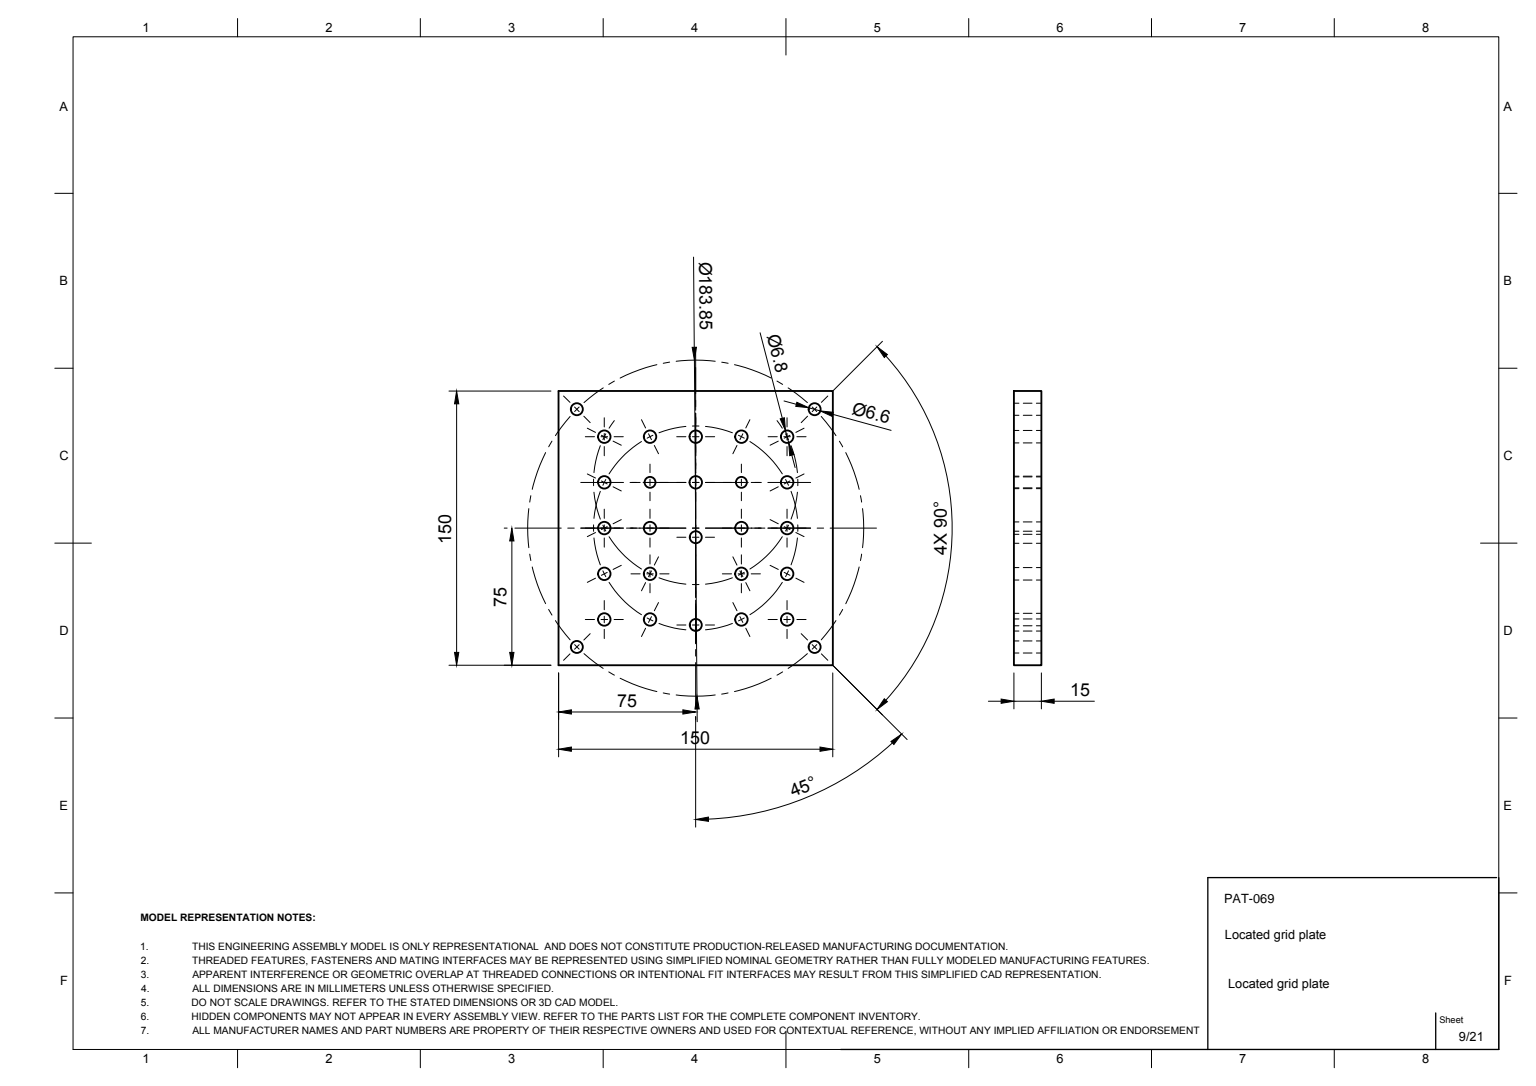
ISO-10303-21;
HEADER;
/* Generated by software containing ST-Developer
 * from STEP Tools, Inc. (www.steptools.com) 
 */

FILE_DESCRIPTION(
/* description */ ('Located fixture plate with toggle clamp'),
/* implementation_level */ '2;1');

FILE_NAME(
/* name */ 'Located grid plate.step',
/* time_stamp */ '2026-10-27T21:36:12-07:00',
/* author */ (''),
/* organization */ (''),
/* preprocessor_version */ 'ST-DEVELOPER v20.2',
/* originating_system */ 'Autodesk Translation Framework v15.17.0.0',
/* authorisation */ '');

FILE_SCHEMA (('AUTOMOTIVE_DESIGN { 1 0 10303 214 3 1 1 }'));
ENDSEC;

DATA;
#10=MECHANICAL_DESIGN_GEOMETRIC_PRESENTATION_REPRESENTATION('',(#325),#9285);
#277=SHAPE_REPRESENTATION_RELATIONSHIP('SRR','None',#9400,#301);
#301=ADVANCED_BREP_SHAPE_REPRESENTATION('',(#348),#9262);
#325=STYLED_ITEM('',(#9598),#348);
#348=MANIFOLD_SOLID_BREP('Body1',#5174);
#388=FACE_BOUND('',#1098,.T.);
#389=FACE_BOUND('',#1099,.T.);
#390=FACE_BOUND('',#1100,.T.);
#391=FACE_BOUND('',#1101,.T.);
#392=FACE_BOUND('',#1102,.T.);
#393=FACE_BOUND('',#1103,.T.);
#394=FACE_BOUND('',#1104,.T.);
#395=FACE_BOUND('',#1105,.T.);
#396=FACE_BOUND('',#1106,.T.);
#397=FACE_BOUND('',#1107,.T.);
#398=FACE_BOUND('',#1108,.T.);
#399=FACE_BOUND('',#1109,.T.);
#400=FACE_BOUND('',#1110,.T.);
#401=FACE_BOUND('',#1111,.T.);
#402=FACE_BOUND('',#1112,.T.);
#403=FACE_BOUND('',#1113,.T.);
#404=FACE_BOUND('',#1114,.T.);
#405=FACE_BOUND('',#1115,.T.);
#406=FACE_BOUND('',#1116,.T.);
#407=FACE_BOUND('',#1117,.T.);
#408=FACE_BOUND('',#1118,.T.);
#409=FACE_BOUND('',#1119,.T.);
#410=FACE_BOUND('',#1120,.T.);
#411=FACE_BOUND('',#1121,.T.);
#412=FACE_BOUND('',#1122,.T.);
#413=FACE_BOUND('',#1123,.T.);
#414=FACE_BOUND('',#1124,.T.);
#415=FACE_BOUND('',#1125,.T.);
#416=FACE_BOUND('',#1128,.T.);
#417=FACE_BOUND('',#1129,.T.);
#418=FACE_BOUND('',#1130,.T.);
#419=FACE_BOUND('',#1131,.T.);
#420=FACE_BOUND('',#1132,.T.);
#421=FACE_BOUND('',#1133,.T.);
#422=FACE_BOUND('',#1134,.T.);
#423=FACE_BOUND('',#1135,.T.);
#424=FACE_BOUND('',#1136,.T.);
#425=FACE_BOUND('',#1137,.T.);
#426=FACE_BOUND('',#1138,.T.);
#427=FACE_BOUND('',#1139,.T.);
#428=FACE_BOUND('',#1140,.T.);
#429=FACE_BOUND('',#1141,.T.);
#430=FACE_BOUND('',#1142,.T.);
#431=FACE_BOUND('',#1143,.T.);
#432=FACE_BOUND('',#1144,.T.);
#433=FACE_BOUND('',#1145,.T.);
#434=FACE_BOUND('',#1146,.T.);
#435=FACE_BOUND('',#1147,.T.);
#436=FACE_BOUND('',#1148,.T.);
#437=FACE_BOUND('',#1149,.T.);
#438=FACE_BOUND('',#1150,.T.);
#439=FACE_BOUND('',#1151,.T.);
#440=FACE_BOUND('',#1152,.T.);
#441=FACE_BOUND('',#1153,.T.);
#442=FACE_BOUND('',#1154,.T.);
#443=FACE_BOUND('',#1155,.T.);
#545=PLANE('',#5666);
#546=PLANE('',#5667);
#547=PLANE('',#5668);
#548=PLANE('',#5669);
#549=PLANE('',#5670);
#550=PLANE('',#5671);
#751=FACE_OUTER_BOUND('',#1068,.T.);
#752=FACE_OUTER_BOUND('',#1069,.T.);
#753=FACE_OUTER_BOUND('',#1070,.T.);
#754=FACE_OUTER_BOUND('',#1071,.T.);
#755=FACE_OUTER_BOUND('',#1072,.T.);
#756=FACE_OUTER_BOUND('',#1073,.T.);
#757=FACE_OUTER_BOUND('',#1074,.T.);
#758=FACE_OUTER_BOUND('',#1075,.T.);
#759=FACE_OUTER_BOUND('',#1076,.T.);
#760=FACE_OUTER_BOUND('',#1077,.T.);
#761=FACE_OUTER_BOUND('',#1078,.T.);
#762=FACE_OUTER_BOUND('',#1079,.T.);
#763=FACE_OUTER_BOUND('',#1080,.T.);
#764=FACE_OUTER_BOUND('',#1081,.T.);
#765=FACE_OUTER_BOUND('',#1082,.T.);
#766=FACE_OUTER_BOUND('',#1083,.T.);
#767=FACE_OUTER_BOUND('',#1084,.T.);
#768=FACE_OUTER_BOUND('',#1085,.T.);
#769=FACE_OUTER_BOUND('',#1086,.T.);
#770=FACE_OUTER_BOUND('',#1087,.T.);
#771=FACE_OUTER_BOUND('',#1088,.T.);
#772=FACE_OUTER_BOUND('',#1089,.T.);
#773=FACE_OUTER_BOUND('',#1090,.T.);
#774=FACE_OUTER_BOUND('',#1091,.T.);
#775=FACE_OUTER_BOUND('',#1092,.T.);
#776=FACE_OUTER_BOUND('',#1093,.T.);
#777=FACE_OUTER_BOUND('',#1094,.T.);
#778=FACE_OUTER_BOUND('',#1095,.T.);
#779=FACE_OUTER_BOUND('',#1096,.T.);
#780=FACE_OUTER_BOUND('',#1097,.T.);
#781=FACE_OUTER_BOUND('',#1126,.T.);
#782=FACE_OUTER_BOUND('',#1127,.T.);
#783=FACE_OUTER_BOUND('',#1156,.T.);
#784=FACE_OUTER_BOUND('',#1157,.T.);
#1068=EDGE_LOOP('',(#3848,#3849,#3850,#3851));
#1069=EDGE_LOOP('',(#3852,#3853,#3854,#3855));
#1070=EDGE_LOOP('',(#3856,#3857,#3858,#3859));
#1071=EDGE_LOOP('',(#3860,#3861,#3862,#3863));
#1072=EDGE_LOOP('',(#3864,#3865,#3866,#3867));
#1073=EDGE_LOOP('',(#3868,#3869,#3870,#3871));
#1074=EDGE_LOOP('',(#3872,#3873,#3874,#3875));
#1075=EDGE_LOOP('',(#3876,#3877,#3878,#3879));
#1076=EDGE_LOOP('',(#3880,#3881,#3882,#3883));
#1077=EDGE_LOOP('',(#3884,#3885,#3886,#3887));
#1078=EDGE_LOOP('',(#3888,#3889,#3890,#3891));
#1079=EDGE_LOOP('',(#3892,#3893,#3894,#3895));
#1080=EDGE_LOOP('',(#3896,#3897,#3898,#3899));
#1081=EDGE_LOOP('',(#3900,#3901,#3902,#3903));
#1082=EDGE_LOOP('',(#3904,#3905,#3906,#3907));
#1083=EDGE_LOOP('',(#3908,#3909,#3910,#3911));
#1084=EDGE_LOOP('',(#3912,#3913,#3914,#3915));
#1085=EDGE_LOOP('',(#3916,#3917,#3918,#3919));
#1086=EDGE_LOOP('',(#3920,#3921,#3922,#3923));
#1087=EDGE_LOOP('',(#3924,#3925,#3926,#3927));
#1088=EDGE_LOOP('',(#3928,#3929,#3930,#3931));
#1089=EDGE_LOOP('',(#3932,#3933,#3934,#3935));
#1090=EDGE_LOOP('',(#3936,#3937,#3938,#3939));
#1091=EDGE_LOOP('',(#3940,#3941,#3942,#3943));
#1092=EDGE_LOOP('',(#3944,#3945,#3946,#3947));
#1093=EDGE_LOOP('',(#3948,#3949,#3950,#3951));
#1094=EDGE_LOOP('',(#3952,#3953,#3954,#3955));
#1095=EDGE_LOOP('',(#3956,#3957,#3958,#3959));
#1096=EDGE_LOOP('',(#3960,#3961,#3962,#3963));
#1097=EDGE_LOOP('',(#3964,#3965,#3966,#3967));
#1098=EDGE_LOOP('',(#3968));
#1099=EDGE_LOOP('',(#3969));
#1100=EDGE_LOOP('',(#3970));
#1101=EDGE_LOOP('',(#3971));
#1102=EDGE_LOOP('',(#3972));
#1103=EDGE_LOOP('',(#3973));
#1104=EDGE_LOOP('',(#3974));
#1105=EDGE_LOOP('',(#3975));
#1106=EDGE_LOOP('',(#3976));
#1107=EDGE_LOOP('',(#3977));
#1108=EDGE_LOOP('',(#3978));
#1109=EDGE_LOOP('',(#3979));
#1110=EDGE_LOOP('',(#3980));
#1111=EDGE_LOOP('',(#3981));
#1112=EDGE_LOOP('',(#3982));
#1113=EDGE_LOOP('',(#3983));
#1114=EDGE_LOOP('',(#3984));
#1115=EDGE_LOOP('',(#3985));
#1116=EDGE_LOOP('',(#3986));
#1117=EDGE_LOOP('',(#3987));
#1118=EDGE_LOOP('',(#3988));
#1119=EDGE_LOOP('',(#3989));
#1120=EDGE_LOOP('',(#3990));
#1121=EDGE_LOOP('',(#3991));
#1122=EDGE_LOOP('',(#3992));
#1123=EDGE_LOOP('',(#3993));
#1124=EDGE_LOOP('',(#3994));
#1125=EDGE_LOOP('',(#3995));
#1126=EDGE_LOOP('',(#3996,#3997,#3998,#3999));
#1127=EDGE_LOOP('',(#4000,#4001,#4002,#4003));
#1128=EDGE_LOOP('',(#4004));
#1129=EDGE_LOOP('',(#4005));
#1130=EDGE_LOOP('',(#4006));
#1131=EDGE_LOOP('',(#4007));
#1132=EDGE_LOOP('',(#4008));
#1133=EDGE_LOOP('',(#4009));
#1134=EDGE_LOOP('',(#4010));
#1135=EDGE_LOOP('',(#4011));
#1136=EDGE_LOOP('',(#4012));
#1137=EDGE_LOOP('',(#4013));
#1138=EDGE_LOOP('',(#4014));
#1139=EDGE_LOOP('',(#4015));
#1140=EDGE_LOOP('',(#4016));
#1141=EDGE_LOOP('',(#4017));
#1142=EDGE_LOOP('',(#4018));
#1143=EDGE_LOOP('',(#4019));
#1144=EDGE_LOOP('',(#4020));
#1145=EDGE_LOOP('',(#4021));
#1146=EDGE_LOOP('',(#4022));
#1147=EDGE_LOOP('',(#4023));
#1148=EDGE_LOOP('',(#4024));
#1149=EDGE_LOOP('',(#4025));
#1150=EDGE_LOOP('',(#4026));
#1151=EDGE_LOOP('',(#4027));
#1152=EDGE_LOOP('',(#4028));
#1153=EDGE_LOOP('',(#4029));
#1154=EDGE_LOOP('',(#4030));
#1155=EDGE_LOOP('',(#4031));
#1156=EDGE_LOOP('',(#4032,#4033,#4034,#4035));
#1157=EDGE_LOOP('',(#4036,#4037,#4038,#4039));
#1419=CIRCLE('',#5583,0.3);
#1420=CIRCLE('',#5584,0.3);
#1421=CIRCLE('',#5586,0.3);
#1422=CIRCLE('',#5587,0.3);
#1423=CIRCLE('',#5589,0.33);
#1424=CIRCLE('',#5590,0.33);
#1425=CIRCLE('',#5592,0.33);
#1426=CIRCLE('',#5593,0.33);
#1427=CIRCLE('',#5595,0.33);
#1428=CIRCLE('',#5596,0.33);
#1429=CIRCLE('',#5598,0.33);
#1430=CIRCLE('',#5599,0.33);
#1431=CIRCLE('',#5601,0.33);
#1432=CIRCLE('',#5602,0.33);
#1433=CIRCLE('',#5604,0.33);
#1434=CIRCLE('',#5605,0.33);
#1435=CIRCLE('',#5607,0.34);
#1436=CIRCLE('',#5608,0.34);
#1437=CIRCLE('',#5610,0.34);
#1438=CIRCLE('',#5611,0.34);
#1439=CIRCLE('',#5613,0.34);
#1440=CIRCLE('',#5614,0.34);
#1441=CIRCLE('',#5616,0.34);
#1442=CIRCLE('',#5617,0.34);
#1443=CIRCLE('',#5619,0.34);
#1444=CIRCLE('',#5620,0.34);
#1445=CIRCLE('',#5622,0.34);
#1446=CIRCLE('',#5623,0.34);
#1447=CIRCLE('',#5625,0.34);
#1448=CIRCLE('',#5626,0.34);
#1449=CIRCLE('',#5628,0.34);
#1450=CIRCLE('',#5629,0.34);
#1451=CIRCLE('',#5631,0.34);
#1452=CIRCLE('',#5632,0.34);
#1453=CIRCLE('',#5634,0.34);
#1454=CIRCLE('',#5635,0.34);
#1455=CIRCLE('',#5637,0.34);
#1456=CIRCLE('',#5638,0.34);
#1457=CIRCLE('',#5640,0.34);
#1458=CIRCLE('',#5641,0.34);
#1459=CIRCLE('',#5643,0.34);
#1460=CIRCLE('',#5644,0.34);
#1461=CIRCLE('',#5646,0.34);
#1462=CIRCLE('',#5647,0.34);
#1463=CIRCLE('',#5649,0.34);
#1464=CIRCLE('',#5650,0.34);
#1465=CIRCLE('',#5652,0.34);
#1466=CIRCLE('',#5653,0.34);
#1467=CIRCLE('',#5655,0.34);
#1468=CIRCLE('',#5656,0.34);
#1469=CIRCLE('',#5658,0.34);
#1470=CIRCLE('',#5659,0.34);
#1471=CIRCLE('',#5661,0.34);
#1472=CIRCLE('',#5662,0.34);
#1473=CIRCLE('',#5664,0.34);
#1474=CIRCLE('',#5665,0.34);
#1727=LINE('',#7966,#2137);
#1728=LINE('',#7972,#2138);
#1729=LINE('',#7978,#2139);
#1730=LINE('',#7984,#2140);
#1731=LINE('',#7990,#2141);
#1732=LINE('',#7996,#2142);
#1733=LINE('',#8002,#2143);
#1734=LINE('',#8008,#2144);
#1735=LINE('',#8014,#2145);
#1736=LINE('',#8020,#2146);
#1737=LINE('',#8026,#2147);
#1738=LINE('',#8032,#2148);
#1739=LINE('',#8038,#2149);
#1740=LINE('',#8044,#2150);
#1741=LINE('',#8050,#2151);
#1742=LINE('',#8056,#2152);
#1743=LINE('',#8062,#2153);
#1744=LINE('',#8068,#2154);
#1745=LINE('',#8074,#2155);
#1746=LINE('',#8080,#2156);
#1747=LINE('',#8086,#2157);
#1748=LINE('',#8092,#2158);
#1749=LINE('',#8098,#2159);
#1750=LINE('',#8104,#2160);
#1751=LINE('',#8110,#2161);
#1752=LINE('',#8116,#2162);
#1753=LINE('',#8122,#2163);
#1754=LINE('',#8128,#2164);
#1755=LINE('',#8133,#2165);
#1756=LINE('',#8135,#2166);
#1757=LINE('',#8137,#2167);
#1758=LINE('',#8138,#2168);
#1759=LINE('',#8141,#2169);
#1760=LINE('',#8143,#2170);
#1761=LINE('',#8144,#2171);
#1762=LINE('',#8147,#2172);
#1763=LINE('',#8149,#2173);
#1764=LINE('',#8150,#2174);
#1765=LINE('',#8152,#2175);
#1766=LINE('',#8153,#2176);
#2137=VECTOR('',#6421,0.3);
#2138=VECTOR('',#6428,0.3);
#2139=VECTOR('',#6435,0.33);
#2140=VECTOR('',#6442,0.33);
#2141=VECTOR('',#6449,0.33);
#2142=VECTOR('',#6456,0.33);
#2143=VECTOR('',#6463,0.33);
#2144=VECTOR('',#6470,0.33);
#2145=VECTOR('',#6477,0.34);
#2146=VECTOR('',#6484,0.34);
#2147=VECTOR('',#6491,0.34);
#2148=VECTOR('',#6498,0.34);
#2149=VECTOR('',#6505,0.34);
#2150=VECTOR('',#6512,0.34);
#2151=VECTOR('',#6519,0.34);
#2152=VECTOR('',#6526,0.34);
#2153=VECTOR('',#6533,0.34);
#2154=VECTOR('',#6540,0.34);
#2155=VECTOR('',#6547,0.34);
#2156=VECTOR('',#6554,0.34);
#2157=VECTOR('',#6561,0.34);
#2158=VECTOR('',#6568,0.34);
#2159=VECTOR('',#6575,0.34);
#2160=VECTOR('',#6582,0.34);
#2161=VECTOR('',#6589,0.34);
#2162=VECTOR('',#6596,0.34);
#2163=VECTOR('',#6603,0.34);
#2164=VECTOR('',#6610,0.34);
#2165=VECTOR('',#6615,1.);
#2166=VECTOR('',#6616,1.);
#2167=VECTOR('',#6617,1.);
#2168=VECTOR('',#6618,1.);
#2169=VECTOR('',#6621,1.);
#2170=VECTOR('',#6622,1.);
#2171=VECTOR('',#6623,1.);
#2172=VECTOR('',#6626,1.);
#2173=VECTOR('',#6627,1.);
#2174=VECTOR('',#6628,1.);
#2175=VECTOR('',#6631,1.);
#2176=VECTOR('',#6632,1.);
#2521=VERTEX_POINT('',#7963);
#2522=VERTEX_POINT('',#7965);
#2523=VERTEX_POINT('',#7969);
#2524=VERTEX_POINT('',#7971);
#2525=VERTEX_POINT('',#7975);
#2526=VERTEX_POINT('',#7977);
#2527=VERTEX_POINT('',#7981);
#2528=VERTEX_POINT('',#7983);
#2529=VERTEX_POINT('',#7987);
#2530=VERTEX_POINT('',#7989);
#2531=VERTEX_POINT('',#7993);
#2532=VERTEX_POINT('',#7995);
#2533=VERTEX_POINT('',#7999);
#2534=VERTEX_POINT('',#8001);
#2535=VERTEX_POINT('',#8005);
#2536=VERTEX_POINT('',#8007);
#2537=VERTEX_POINT('',#8011);
#2538=VERTEX_POINT('',#8013);
#2539=VERTEX_POINT('',#8017);
#2540=VERTEX_POINT('',#8019);
#2541=VERTEX_POINT('',#8023);
#2542=VERTEX_POINT('',#8025);
#2543=VERTEX_POINT('',#8029);
#2544=VERTEX_POINT('',#8031);
#2545=VERTEX_POINT('',#8035);
#2546=VERTEX_POINT('',#8037);
#2547=VERTEX_POINT('',#8041);
#2548=VERTEX_POINT('',#8043);
#2549=VERTEX_POINT('',#8047);
#2550=VERTEX_POINT('',#8049);
#2551=VERTEX_POINT('',#8053);
#2552=VERTEX_POINT('',#8055);
#2553=VERTEX_POINT('',#8059);
#2554=VERTEX_POINT('',#8061);
#2555=VERTEX_POINT('',#8065);
#2556=VERTEX_POINT('',#8067);
#2557=VERTEX_POINT('',#8071);
#2558=VERTEX_POINT('',#8073);
#2559=VERTEX_POINT('',#8077);
#2560=VERTEX_POINT('',#8079);
#2561=VERTEX_POINT('',#8083);
#2562=VERTEX_POINT('',#8085);
#2563=VERTEX_POINT('',#8089);
#2564=VERTEX_POINT('',#8091);
#2565=VERTEX_POINT('',#8095);
#2566=VERTEX_POINT('',#8097);
#2567=VERTEX_POINT('',#8101);
#2568=VERTEX_POINT('',#8103);
#2569=VERTEX_POINT('',#8107);
#2570=VERTEX_POINT('',#8109);
#2571=VERTEX_POINT('',#8113);
#2572=VERTEX_POINT('',#8115);
#2573=VERTEX_POINT('',#8119);
#2574=VERTEX_POINT('',#8121);
#2575=VERTEX_POINT('',#8125);
#2576=VERTEX_POINT('',#8127);
#2577=VERTEX_POINT('',#8131);
#2578=VERTEX_POINT('',#8132);
#2579=VERTEX_POINT('',#8134);
#2580=VERTEX_POINT('',#8136);
#2581=VERTEX_POINT('',#8140);
#2582=VERTEX_POINT('',#8142);
#2583=VERTEX_POINT('',#8146);
#2584=VERTEX_POINT('',#8148);
#3012=EDGE_CURVE('',#2521,#2521,#1419,.T.);
#3013=EDGE_CURVE('',#2521,#2522,#1727,.T.);
#3014=EDGE_CURVE('',#2522,#2522,#1420,.T.);
#3015=EDGE_CURVE('',#2523,#2523,#1421,.T.);
#3016=EDGE_CURVE('',#2523,#2524,#1728,.T.);
#3017=EDGE_CURVE('',#2524,#2524,#1422,.T.);
#3018=EDGE_CURVE('',#2525,#2525,#1423,.T.);
#3019=EDGE_CURVE('',#2525,#2526,#1729,.T.);
#3020=EDGE_CURVE('',#2526,#2526,#1424,.T.);
#3021=EDGE_CURVE('',#2527,#2527,#1425,.T.);
#3022=EDGE_CURVE('',#2527,#2528,#1730,.T.);
#3023=EDGE_CURVE('',#2528,#2528,#1426,.T.);
#3024=EDGE_CURVE('',#2529,#2529,#1427,.T.);
#3025=EDGE_CURVE('',#2529,#2530,#1731,.T.);
#3026=EDGE_CURVE('',#2530,#2530,#1428,.T.);
#3027=EDGE_CURVE('',#2531,#2531,#1429,.T.);
#3028=EDGE_CURVE('',#2531,#2532,#1732,.T.);
#3029=EDGE_CURVE('',#2532,#2532,#1430,.T.);
#3030=EDGE_CURVE('',#2533,#2533,#1431,.T.);
#3031=EDGE_CURVE('',#2533,#2534,#1733,.T.);
#3032=EDGE_CURVE('',#2534,#2534,#1432,.T.);
#3033=EDGE_CURVE('',#2535,#2535,#1433,.T.);
#3034=EDGE_CURVE('',#2535,#2536,#1734,.T.);
#3035=EDGE_CURVE('',#2536,#2536,#1434,.T.);
#3036=EDGE_CURVE('',#2537,#2537,#1435,.T.);
#3037=EDGE_CURVE('',#2537,#2538,#1735,.T.);
#3038=EDGE_CURVE('',#2538,#2538,#1436,.T.);
#3039=EDGE_CURVE('',#2539,#2539,#1437,.T.);
#3040=EDGE_CURVE('',#2539,#2540,#1736,.T.);
#3041=EDGE_CURVE('',#2540,#2540,#1438,.T.);
#3042=EDGE_CURVE('',#2541,#2541,#1439,.T.);
#3043=EDGE_CURVE('',#2541,#2542,#1737,.T.);
#3044=EDGE_CURVE('',#2542,#2542,#1440,.T.);
#3045=EDGE_CURVE('',#2543,#2543,#1441,.T.);
#3046=EDGE_CURVE('',#2543,#2544,#1738,.T.);
#3047=EDGE_CURVE('',#2544,#2544,#1442,.T.);
#3048=EDGE_CURVE('',#2545,#2545,#1443,.T.);
#3049=EDGE_CURVE('',#2545,#2546,#1739,.T.);
#3050=EDGE_CURVE('',#2546,#2546,#1444,.T.);
#3051=EDGE_CURVE('',#2547,#2547,#1445,.T.);
#3052=EDGE_CURVE('',#2547,#2548,#1740,.T.);
#3053=EDGE_CURVE('',#2548,#2548,#1446,.T.);
#3054=EDGE_CURVE('',#2549,#2549,#1447,.T.);
#3055=EDGE_CURVE('',#2549,#2550,#1741,.T.);
#3056=EDGE_CURVE('',#2550,#2550,#1448,.T.);
#3057=EDGE_CURVE('',#2551,#2551,#1449,.T.);
#3058=EDGE_CURVE('',#2551,#2552,#1742,.T.);
#3059=EDGE_CURVE('',#2552,#2552,#1450,.T.);
#3060=EDGE_CURVE('',#2553,#2553,#1451,.T.);
#3061=EDGE_CURVE('',#2553,#2554,#1743,.T.);
#3062=EDGE_CURVE('',#2554,#2554,#1452,.T.);
#3063=EDGE_CURVE('',#2555,#2555,#1453,.T.);
#3064=EDGE_CURVE('',#2555,#2556,#1744,.T.);
#3065=EDGE_CURVE('',#2556,#2556,#1454,.T.);
#3066=EDGE_CURVE('',#2557,#2557,#1455,.T.);
#3067=EDGE_CURVE('',#2557,#2558,#1745,.T.);
#3068=EDGE_CURVE('',#2558,#2558,#1456,.T.);
#3069=EDGE_CURVE('',#2559,#2559,#1457,.T.);
#3070=EDGE_CURVE('',#2559,#2560,#1746,.T.);
#3071=EDGE_CURVE('',#2560,#2560,#1458,.T.);
#3072=EDGE_CURVE('',#2561,#2561,#1459,.T.);
#3073=EDGE_CURVE('',#2561,#2562,#1747,.T.);
#3074=EDGE_CURVE('',#2562,#2562,#1460,.T.);
#3075=EDGE_CURVE('',#2563,#2563,#1461,.T.);
#3076=EDGE_CURVE('',#2563,#2564,#1748,.T.);
#3077=EDGE_CURVE('',#2564,#2564,#1462,.T.);
#3078=EDGE_CURVE('',#2565,#2565,#1463,.T.);
#3079=EDGE_CURVE('',#2565,#2566,#1749,.T.);
#3080=EDGE_CURVE('',#2566,#2566,#1464,.T.);
#3081=EDGE_CURVE('',#2567,#2567,#1465,.T.);
#3082=EDGE_CURVE('',#2567,#2568,#1750,.T.);
#3083=EDGE_CURVE('',#2568,#2568,#1466,.T.);
#3084=EDGE_CURVE('',#2569,#2569,#1467,.T.);
#3085=EDGE_CURVE('',#2569,#2570,#1751,.T.);
#3086=EDGE_CURVE('',#2570,#2570,#1468,.T.);
#3087=EDGE_CURVE('',#2571,#2571,#1469,.T.);
#3088=EDGE_CURVE('',#2571,#2572,#1752,.T.);
#3089=EDGE_CURVE('',#2572,#2572,#1470,.T.);
#3090=EDGE_CURVE('',#2573,#2573,#1471,.T.);
#3091=EDGE_CURVE('',#2573,#2574,#1753,.T.);
#3092=EDGE_CURVE('',#2574,#2574,#1472,.T.);
#3093=EDGE_CURVE('',#2575,#2575,#1473,.T.);
#3094=EDGE_CURVE('',#2575,#2576,#1754,.T.);
#3095=EDGE_CURVE('',#2576,#2576,#1474,.T.);
#3096=EDGE_CURVE('',#2577,#2578,#1755,.T.);
#3097=EDGE_CURVE('',#2578,#2579,#1756,.T.);
#3098=EDGE_CURVE('',#2580,#2579,#1757,.T.);
#3099=EDGE_CURVE('',#2577,#2580,#1758,.T.);
#3100=EDGE_CURVE('',#2581,#2577,#1759,.T.);
#3101=EDGE_CURVE('',#2582,#2580,#1760,.T.);
#3102=EDGE_CURVE('',#2581,#2582,#1761,.T.);
#3103=EDGE_CURVE('',#2583,#2581,#1762,.T.);
#3104=EDGE_CURVE('',#2584,#2582,#1763,.T.);
#3105=EDGE_CURVE('',#2583,#2584,#1764,.T.);
#3106=EDGE_CURVE('',#2578,#2583,#1765,.T.);
#3107=EDGE_CURVE('',#2579,#2584,#1766,.T.);
#3848=ORIENTED_EDGE('',*,*,#3012,.F.);
#3849=ORIENTED_EDGE('',*,*,#3013,.T.);
#3850=ORIENTED_EDGE('',*,*,#3014,.F.);
#3851=ORIENTED_EDGE('',*,*,#3013,.F.);
#3852=ORIENTED_EDGE('',*,*,#3015,.F.);
#3853=ORIENTED_EDGE('',*,*,#3016,.T.);
#3854=ORIENTED_EDGE('',*,*,#3017,.F.);
#3855=ORIENTED_EDGE('',*,*,#3016,.F.);
#3856=ORIENTED_EDGE('',*,*,#3018,.F.);
#3857=ORIENTED_EDGE('',*,*,#3019,.T.);
#3858=ORIENTED_EDGE('',*,*,#3020,.F.);
#3859=ORIENTED_EDGE('',*,*,#3019,.F.);
#3860=ORIENTED_EDGE('',*,*,#3021,.F.);
#3861=ORIENTED_EDGE('',*,*,#3022,.T.);
#3862=ORIENTED_EDGE('',*,*,#3023,.F.);
#3863=ORIENTED_EDGE('',*,*,#3022,.F.);
#3864=ORIENTED_EDGE('',*,*,#3024,.F.);
#3865=ORIENTED_EDGE('',*,*,#3025,.T.);
#3866=ORIENTED_EDGE('',*,*,#3026,.F.);
#3867=ORIENTED_EDGE('',*,*,#3025,.F.);
#3868=ORIENTED_EDGE('',*,*,#3027,.F.);
#3869=ORIENTED_EDGE('',*,*,#3028,.T.);
#3870=ORIENTED_EDGE('',*,*,#3029,.F.);
#3871=ORIENTED_EDGE('',*,*,#3028,.F.);
#3872=ORIENTED_EDGE('',*,*,#3030,.F.);
#3873=ORIENTED_EDGE('',*,*,#3031,.T.);
#3874=ORIENTED_EDGE('',*,*,#3032,.F.);
#3875=ORIENTED_EDGE('',*,*,#3031,.F.);
#3876=ORIENTED_EDGE('',*,*,#3033,.F.);
#3877=ORIENTED_EDGE('',*,*,#3034,.T.);
#3878=ORIENTED_EDGE('',*,*,#3035,.F.);
#3879=ORIENTED_EDGE('',*,*,#3034,.F.);
#3880=ORIENTED_EDGE('',*,*,#3036,.F.);
#3881=ORIENTED_EDGE('',*,*,#3037,.T.);
#3882=ORIENTED_EDGE('',*,*,#3038,.F.);
#3883=ORIENTED_EDGE('',*,*,#3037,.F.);
#3884=ORIENTED_EDGE('',*,*,#3039,.F.);
#3885=ORIENTED_EDGE('',*,*,#3040,.T.);
#3886=ORIENTED_EDGE('',*,*,#3041,.F.);
#3887=ORIENTED_EDGE('',*,*,#3040,.F.);
#3888=ORIENTED_EDGE('',*,*,#3042,.F.);
#3889=ORIENTED_EDGE('',*,*,#3043,.T.);
#3890=ORIENTED_EDGE('',*,*,#3044,.F.);
#3891=ORIENTED_EDGE('',*,*,#3043,.F.);
#3892=ORIENTED_EDGE('',*,*,#3045,.F.);
#3893=ORIENTED_EDGE('',*,*,#3046,.T.);
#3894=ORIENTED_EDGE('',*,*,#3047,.F.);
#3895=ORIENTED_EDGE('',*,*,#3046,.F.);
#3896=ORIENTED_EDGE('',*,*,#3048,.F.);
#3897=ORIENTED_EDGE('',*,*,#3049,.T.);
#3898=ORIENTED_EDGE('',*,*,#3050,.F.);
#3899=ORIENTED_EDGE('',*,*,#3049,.F.);
#3900=ORIENTED_EDGE('',*,*,#3051,.F.);
#3901=ORIENTED_EDGE('',*,*,#3052,.T.);
#3902=ORIENTED_EDGE('',*,*,#3053,.F.);
#3903=ORIENTED_EDGE('',*,*,#3052,.F.);
#3904=ORIENTED_EDGE('',*,*,#3054,.F.);
#3905=ORIENTED_EDGE('',*,*,#3055,.T.);
#3906=ORIENTED_EDGE('',*,*,#3056,.F.);
#3907=ORIENTED_EDGE('',*,*,#3055,.F.);
#3908=ORIENTED_EDGE('',*,*,#3057,.F.);
#3909=ORIENTED_EDGE('',*,*,#3058,.T.);
#3910=ORIENTED_EDGE('',*,*,#3059,.F.);
#3911=ORIENTED_EDGE('',*,*,#3058,.F.);
#3912=ORIENTED_EDGE('',*,*,#3060,.F.);
#3913=ORIENTED_EDGE('',*,*,#3061,.T.);
#3914=ORIENTED_EDGE('',*,*,#3062,.F.);
#3915=ORIENTED_EDGE('',*,*,#3061,.F.);
#3916=ORIENTED_EDGE('',*,*,#3063,.F.);
#3917=ORIENTED_EDGE('',*,*,#3064,.T.);
#3918=ORIENTED_EDGE('',*,*,#3065,.F.);
#3919=ORIENTED_EDGE('',*,*,#3064,.F.);
#3920=ORIENTED_EDGE('',*,*,#3066,.F.);
#3921=ORIENTED_EDGE('',*,*,#3067,.T.);
#3922=ORIENTED_EDGE('',*,*,#3068,.F.);
#3923=ORIENTED_EDGE('',*,*,#3067,.F.);
#3924=ORIENTED_EDGE('',*,*,#3069,.F.);
#3925=ORIENTED_EDGE('',*,*,#3070,.T.);
#3926=ORIENTED_EDGE('',*,*,#3071,.F.);
#3927=ORIENTED_EDGE('',*,*,#3070,.F.);
#3928=ORIENTED_EDGE('',*,*,#3072,.F.);
#3929=ORIENTED_EDGE('',*,*,#3073,.T.);
#3930=ORIENTED_EDGE('',*,*,#3074,.F.);
#3931=ORIENTED_EDGE('',*,*,#3073,.F.);
#3932=ORIENTED_EDGE('',*,*,#3075,.F.);
#3933=ORIENTED_EDGE('',*,*,#3076,.T.);
#3934=ORIENTED_EDGE('',*,*,#3077,.F.);
#3935=ORIENTED_EDGE('',*,*,#3076,.F.);
#3936=ORIENTED_EDGE('',*,*,#3078,.F.);
#3937=ORIENTED_EDGE('',*,*,#3079,.T.);
#3938=ORIENTED_EDGE('',*,*,#3080,.F.);
#3939=ORIENTED_EDGE('',*,*,#3079,.F.);
#3940=ORIENTED_EDGE('',*,*,#3081,.F.);
#3941=ORIENTED_EDGE('',*,*,#3082,.T.);
#3942=ORIENTED_EDGE('',*,*,#3083,.F.);
#3943=ORIENTED_EDGE('',*,*,#3082,.F.);
#3944=ORIENTED_EDGE('',*,*,#3084,.F.);
#3945=ORIENTED_EDGE('',*,*,#3085,.T.);
#3946=ORIENTED_EDGE('',*,*,#3086,.F.);
#3947=ORIENTED_EDGE('',*,*,#3085,.F.);
#3948=ORIENTED_EDGE('',*,*,#3087,.F.);
#3949=ORIENTED_EDGE('',*,*,#3088,.T.);
#3950=ORIENTED_EDGE('',*,*,#3089,.F.);
#3951=ORIENTED_EDGE('',*,*,#3088,.F.);
#3952=ORIENTED_EDGE('',*,*,#3090,.F.);
#3953=ORIENTED_EDGE('',*,*,#3091,.T.);
#3954=ORIENTED_EDGE('',*,*,#3092,.F.);
#3955=ORIENTED_EDGE('',*,*,#3091,.F.);
#3956=ORIENTED_EDGE('',*,*,#3093,.F.);
#3957=ORIENTED_EDGE('',*,*,#3094,.T.);
#3958=ORIENTED_EDGE('',*,*,#3095,.F.);
#3959=ORIENTED_EDGE('',*,*,#3094,.F.);
#3960=ORIENTED_EDGE('',*,*,#3096,.T.);
#3961=ORIENTED_EDGE('',*,*,#3097,.T.);
#3962=ORIENTED_EDGE('',*,*,#3098,.F.);
#3963=ORIENTED_EDGE('',*,*,#3099,.F.);
#3964=ORIENTED_EDGE('',*,*,#3100,.T.);
#3965=ORIENTED_EDGE('',*,*,#3099,.T.);
#3966=ORIENTED_EDGE('',*,*,#3101,.F.);
#3967=ORIENTED_EDGE('',*,*,#3102,.F.);
#3968=ORIENTED_EDGE('',*,*,#3020,.T.);
#3969=ORIENTED_EDGE('',*,*,#3023,.T.);
#3970=ORIENTED_EDGE('',*,*,#3026,.T.);
#3971=ORIENTED_EDGE('',*,*,#3029,.T.);
#3972=ORIENTED_EDGE('',*,*,#3038,.T.);
#3973=ORIENTED_EDGE('',*,*,#3041,.T.);
#3974=ORIENTED_EDGE('',*,*,#3044,.T.);
#3975=ORIENTED_EDGE('',*,*,#3047,.T.);
#3976=ORIENTED_EDGE('',*,*,#3050,.T.);
#3977=ORIENTED_EDGE('',*,*,#3053,.T.);
#3978=ORIENTED_EDGE('',*,*,#3056,.T.);
#3979=ORIENTED_EDGE('',*,*,#3059,.T.);
#3980=ORIENTED_EDGE('',*,*,#3062,.T.);
#3981=ORIENTED_EDGE('',*,*,#3065,.T.);
#3982=ORIENTED_EDGE('',*,*,#3068,.T.);
#3983=ORIENTED_EDGE('',*,*,#3071,.T.);
#3984=ORIENTED_EDGE('',*,*,#3074,.T.);
#3985=ORIENTED_EDGE('',*,*,#3077,.T.);
#3986=ORIENTED_EDGE('',*,*,#3080,.T.);
#3987=ORIENTED_EDGE('',*,*,#3083,.T.);
#3988=ORIENTED_EDGE('',*,*,#3086,.T.);
#3989=ORIENTED_EDGE('',*,*,#3089,.T.);
#3990=ORIENTED_EDGE('',*,*,#3092,.T.);
#3991=ORIENTED_EDGE('',*,*,#3095,.T.);
#3992=ORIENTED_EDGE('',*,*,#3035,.T.);
#3993=ORIENTED_EDGE('',*,*,#3032,.T.);
#3994=ORIENTED_EDGE('',*,*,#3017,.T.);
#3995=ORIENTED_EDGE('',*,*,#3014,.T.);
#3996=ORIENTED_EDGE('',*,*,#3103,.T.);
#3997=ORIENTED_EDGE('',*,*,#3102,.T.);
#3998=ORIENTED_EDGE('',*,*,#3104,.F.);
#3999=ORIENTED_EDGE('',*,*,#3105,.F.);
#4000=ORIENTED_EDGE('',*,*,#3106,.T.);
#4001=ORIENTED_EDGE('',*,*,#3105,.T.);
#4002=ORIENTED_EDGE('',*,*,#3107,.F.);
#4003=ORIENTED_EDGE('',*,*,#3097,.F.);
#4004=ORIENTED_EDGE('',*,*,#3018,.T.);
#4005=ORIENTED_EDGE('',*,*,#3021,.T.);
#4006=ORIENTED_EDGE('',*,*,#3024,.T.);
#4007=ORIENTED_EDGE('',*,*,#3027,.T.);
#4008=ORIENTED_EDGE('',*,*,#3036,.T.);
#4009=ORIENTED_EDGE('',*,*,#3039,.T.);
#4010=ORIENTED_EDGE('',*,*,#3042,.T.);
#4011=ORIENTED_EDGE('',*,*,#3045,.T.);
#4012=ORIENTED_EDGE('',*,*,#3048,.T.);
#4013=ORIENTED_EDGE('',*,*,#3051,.T.);
#4014=ORIENTED_EDGE('',*,*,#3054,.T.);
#4015=ORIENTED_EDGE('',*,*,#3057,.T.);
#4016=ORIENTED_EDGE('',*,*,#3060,.T.);
#4017=ORIENTED_EDGE('',*,*,#3063,.T.);
#4018=ORIENTED_EDGE('',*,*,#3066,.T.);
#4019=ORIENTED_EDGE('',*,*,#3069,.T.);
#4020=ORIENTED_EDGE('',*,*,#3072,.T.);
#4021=ORIENTED_EDGE('',*,*,#3075,.T.);
#4022=ORIENTED_EDGE('',*,*,#3078,.T.);
#4023=ORIENTED_EDGE('',*,*,#3081,.T.);
#4024=ORIENTED_EDGE('',*,*,#3084,.T.);
#4025=ORIENTED_EDGE('',*,*,#3087,.T.);
#4026=ORIENTED_EDGE('',*,*,#3090,.T.);
#4027=ORIENTED_EDGE('',*,*,#3093,.T.);
#4028=ORIENTED_EDGE('',*,*,#3033,.T.);
#4029=ORIENTED_EDGE('',*,*,#3030,.T.);
#4030=ORIENTED_EDGE('',*,*,#3015,.T.);
#4031=ORIENTED_EDGE('',*,*,#3012,.T.);
#4032=ORIENTED_EDGE('',*,*,#3107,.T.);
#4033=ORIENTED_EDGE('',*,*,#3104,.T.);
#4034=ORIENTED_EDGE('',*,*,#3101,.T.);
#4035=ORIENTED_EDGE('',*,*,#3098,.T.);
#4036=ORIENTED_EDGE('',*,*,#3106,.F.);
#4037=ORIENTED_EDGE('',*,*,#3096,.F.);
#4038=ORIENTED_EDGE('',*,*,#3100,.F.);
#4039=ORIENTED_EDGE('',*,*,#3103,.F.);
#4807=CYLINDRICAL_SURFACE('',#5582,0.3);
#4808=CYLINDRICAL_SURFACE('',#5585,0.3);
#4809=CYLINDRICAL_SURFACE('',#5588,0.33);
#4810=CYLINDRICAL_SURFACE('',#5591,0.33);
#4811=CYLINDRICAL_SURFACE('',#5594,0.33);
#4812=CYLINDRICAL_SURFACE('',#5597,0.33);
#4813=CYLINDRICAL_SURFACE('',#5600,0.33);
#4814=CYLINDRICAL_SURFACE('',#5603,0.33);
#4815=CYLINDRICAL_SURFACE('',#5606,0.34);
#4816=CYLINDRICAL_SURFACE('',#5609,0.34);
#4817=CYLINDRICAL_SURFACE('',#5612,0.34);
#4818=CYLINDRICAL_SURFACE('',#5615,0.34);
#4819=CYLINDRICAL_SURFACE('',#5618,0.34);
#4820=CYLINDRICAL_SURFACE('',#5621,0.34);
#4821=CYLINDRICAL_SURFACE('',#5624,0.34);
#4822=CYLINDRICAL_SURFACE('',#5627,0.34);
#4823=CYLINDRICAL_SURFACE('',#5630,0.34);
#4824=CYLINDRICAL_SURFACE('',#5633,0.34);
#4825=CYLINDRICAL_SURFACE('',#5636,0.34);
#4826=CYLINDRICAL_SURFACE('',#5639,0.34);
#4827=CYLINDRICAL_SURFACE('',#5642,0.34);
#4828=CYLINDRICAL_SURFACE('',#5645,0.34);
#4829=CYLINDRICAL_SURFACE('',#5648,0.34);
#4830=CYLINDRICAL_SURFACE('',#5651,0.34);
#4831=CYLINDRICAL_SURFACE('',#5654,0.34);
#4832=CYLINDRICAL_SURFACE('',#5657,0.34);
#4833=CYLINDRICAL_SURFACE('',#5660,0.34);
#4834=CYLINDRICAL_SURFACE('',#5663,0.34);
#4952=ADVANCED_FACE('',(#751),#4807,.F.);
#4953=ADVANCED_FACE('',(#752),#4808,.F.);
#4954=ADVANCED_FACE('',(#753),#4809,.F.);
#4955=ADVANCED_FACE('',(#754),#4810,.F.);
#4956=ADVANCED_FACE('',(#755),#4811,.F.);
#4957=ADVANCED_FACE('',(#756),#4812,.F.);
#4958=ADVANCED_FACE('',(#757),#4813,.F.);
#4959=ADVANCED_FACE('',(#758),#4814,.F.);
#4960=ADVANCED_FACE('',(#759),#4815,.F.);
#4961=ADVANCED_FACE('',(#760),#4816,.F.);
#4962=ADVANCED_FACE('',(#761),#4817,.F.);
#4963=ADVANCED_FACE('',(#762),#4818,.F.);
#4964=ADVANCED_FACE('',(#763),#4819,.F.);
#4965=ADVANCED_FACE('',(#764),#4820,.F.);
#4966=ADVANCED_FACE('',(#765),#4821,.F.);
#4967=ADVANCED_FACE('',(#766),#4822,.F.);
#4968=ADVANCED_FACE('',(#767),#4823,.F.);
#4969=ADVANCED_FACE('',(#768),#4824,.F.);
#4970=ADVANCED_FACE('',(#769),#4825,.F.);
#4971=ADVANCED_FACE('',(#770),#4826,.F.);
#4972=ADVANCED_FACE('',(#771),#4827,.F.);
#4973=ADVANCED_FACE('',(#772),#4828,.F.);
#4974=ADVANCED_FACE('',(#773),#4829,.F.);
#4975=ADVANCED_FACE('',(#774),#4830,.F.);
#4976=ADVANCED_FACE('',(#775),#4831,.F.);
#4977=ADVANCED_FACE('',(#776),#4832,.F.);
#4978=ADVANCED_FACE('',(#777),#4833,.F.);
#4979=ADVANCED_FACE('',(#778),#4834,.F.);
#4980=ADVANCED_FACE('',(#779),#545,.T.);
#4981=ADVANCED_FACE('',(#780,#388,#389,#390,#391,#392,#393,#394,#395,#396,
#397,#398,#399,#400,#401,#402,#403,#404,#405,#406,#407,#408,#409,#410,#411,
#412,#413,#414,#415),#546,.T.);
#4982=ADVANCED_FACE('',(#781),#547,.T.);
#4983=ADVANCED_FACE('',(#782,#416,#417,#418,#419,#420,#421,#422,#423,#424,
#425,#426,#427,#428,#429,#430,#431,#432,#433,#434,#435,#436,#437,#438,#439,
#440,#441,#442,#443),#548,.T.);
#4984=ADVANCED_FACE('',(#783),#549,.T.);
#4985=ADVANCED_FACE('',(#784),#550,.F.);
#5174=CLOSED_SHELL('',(#4952,#4953,#4954,#4955,#4956,#4957,#4958,#4959,
#4960,#4961,#4962,#4963,#4964,#4965,#4966,#4967,#4968,#4969,#4970,#4971,
#4972,#4973,#4974,#4975,#4976,#4977,#4978,#4979,#4980,#4981,#4982,#4983,
#4984,#4985));
#5581=AXIS2_PLACEMENT_3D('',#7961,#6415,#6416);
#5582=AXIS2_PLACEMENT_3D('',#7962,#6417,#6418);
#5583=AXIS2_PLACEMENT_3D('',#7964,#6419,#6420);
#5584=AXIS2_PLACEMENT_3D('',#7967,#6422,#6423);
#5585=AXIS2_PLACEMENT_3D('',#7968,#6424,#6425);
#5586=AXIS2_PLACEMENT_3D('',#7970,#6426,#6427);
#5587=AXIS2_PLACEMENT_3D('',#7973,#6429,#6430);
#5588=AXIS2_PLACEMENT_3D('',#7974,#6431,#6432);
#5589=AXIS2_PLACEMENT_3D('',#7976,#6433,#6434);
#5590=AXIS2_PLACEMENT_3D('',#7979,#6436,#6437);
#5591=AXIS2_PLACEMENT_3D('',#7980,#6438,#6439);
#5592=AXIS2_PLACEMENT_3D('',#7982,#6440,#6441);
#5593=AXIS2_PLACEMENT_3D('',#7985,#6443,#6444);
#5594=AXIS2_PLACEMENT_3D('',#7986,#6445,#6446);
#5595=AXIS2_PLACEMENT_3D('',#7988,#6447,#6448);
#5596=AXIS2_PLACEMENT_3D('',#7991,#6450,#6451);
#5597=AXIS2_PLACEMENT_3D('',#7992,#6452,#6453);
#5598=AXIS2_PLACEMENT_3D('',#7994,#6454,#6455);
#5599=AXIS2_PLACEMENT_3D('',#7997,#6457,#6458);
#5600=AXIS2_PLACEMENT_3D('',#7998,#6459,#6460);
#5601=AXIS2_PLACEMENT_3D('',#8000,#6461,#6462);
#5602=AXIS2_PLACEMENT_3D('',#8003,#6464,#6465);
#5603=AXIS2_PLACEMENT_3D('',#8004,#6466,#6467);
#5604=AXIS2_PLACEMENT_3D('',#8006,#6468,#6469);
#5605=AXIS2_PLACEMENT_3D('',#8009,#6471,#6472);
#5606=AXIS2_PLACEMENT_3D('',#8010,#6473,#6474);
#5607=AXIS2_PLACEMENT_3D('',#8012,#6475,#6476);
#5608=AXIS2_PLACEMENT_3D('',#8015,#6478,#6479);
#5609=AXIS2_PLACEMENT_3D('',#8016,#6480,#6481);
#5610=AXIS2_PLACEMENT_3D('',#8018,#6482,#6483);
#5611=AXIS2_PLACEMENT_3D('',#8021,#6485,#6486);
#5612=AXIS2_PLACEMENT_3D('',#8022,#6487,#6488);
#5613=AXIS2_PLACEMENT_3D('',#8024,#6489,#6490);
#5614=AXIS2_PLACEMENT_3D('',#8027,#6492,#6493);
#5615=AXIS2_PLACEMENT_3D('',#8028,#6494,#6495);
#5616=AXIS2_PLACEMENT_3D('',#8030,#6496,#6497);
#5617=AXIS2_PLACEMENT_3D('',#8033,#6499,#6500);
#5618=AXIS2_PLACEMENT_3D('',#8034,#6501,#6502);
#5619=AXIS2_PLACEMENT_3D('',#8036,#6503,#6504);
#5620=AXIS2_PLACEMENT_3D('',#8039,#6506,#6507);
#5621=AXIS2_PLACEMENT_3D('',#8040,#6508,#6509);
#5622=AXIS2_PLACEMENT_3D('',#8042,#6510,#6511);
#5623=AXIS2_PLACEMENT_3D('',#8045,#6513,#6514);
#5624=AXIS2_PLACEMENT_3D('',#8046,#6515,#6516);
#5625=AXIS2_PLACEMENT_3D('',#8048,#6517,#6518);
#5626=AXIS2_PLACEMENT_3D('',#8051,#6520,#6521);
#5627=AXIS2_PLACEMENT_3D('',#8052,#6522,#6523);
#5628=AXIS2_PLACEMENT_3D('',#8054,#6524,#6525);
#5629=AXIS2_PLACEMENT_3D('',#8057,#6527,#6528);
#5630=AXIS2_PLACEMENT_3D('',#8058,#6529,#6530);
#5631=AXIS2_PLACEMENT_3D('',#8060,#6531,#6532);
#5632=AXIS2_PLACEMENT_3D('',#8063,#6534,#6535);
#5633=AXIS2_PLACEMENT_3D('',#8064,#6536,#6537);
#5634=AXIS2_PLACEMENT_3D('',#8066,#6538,#6539);
#5635=AXIS2_PLACEMENT_3D('',#8069,#6541,#6542);
#5636=AXIS2_PLACEMENT_3D('',#8070,#6543,#6544);
#5637=AXIS2_PLACEMENT_3D('',#8072,#6545,#6546);
#5638=AXIS2_PLACEMENT_3D('',#8075,#6548,#6549);
#5639=AXIS2_PLACEMENT_3D('',#8076,#6550,#6551);
#5640=AXIS2_PLACEMENT_3D('',#8078,#6552,#6553);
#5641=AXIS2_PLACEMENT_3D('',#8081,#6555,#6556);
#5642=AXIS2_PLACEMENT_3D('',#8082,#6557,#6558);
#5643=AXIS2_PLACEMENT_3D('',#8084,#6559,#6560);
#5644=AXIS2_PLACEMENT_3D('',#8087,#6562,#6563);
#5645=AXIS2_PLACEMENT_3D('',#8088,#6564,#6565);
#5646=AXIS2_PLACEMENT_3D('',#8090,#6566,#6567);
#5647=AXIS2_PLACEMENT_3D('',#8093,#6569,#6570);
#5648=AXIS2_PLACEMENT_3D('',#8094,#6571,#6572);
#5649=AXIS2_PLACEMENT_3D('',#8096,#6573,#6574);
#5650=AXIS2_PLACEMENT_3D('',#8099,#6576,#6577);
#5651=AXIS2_PLACEMENT_3D('',#8100,#6578,#6579);
#5652=AXIS2_PLACEMENT_3D('',#8102,#6580,#6581);
#5653=AXIS2_PLACEMENT_3D('',#8105,#6583,#6584);
#5654=AXIS2_PLACEMENT_3D('',#8106,#6585,#6586);
#5655=AXIS2_PLACEMENT_3D('',#8108,#6587,#6588);
#5656=AXIS2_PLACEMENT_3D('',#8111,#6590,#6591);
#5657=AXIS2_PLACEMENT_3D('',#8112,#6592,#6593);
#5658=AXIS2_PLACEMENT_3D('',#8114,#6594,#6595);
#5659=AXIS2_PLACEMENT_3D('',#8117,#6597,#6598);
#5660=AXIS2_PLACEMENT_3D('',#8118,#6599,#6600);
#5661=AXIS2_PLACEMENT_3D('',#8120,#6601,#6602);
#5662=AXIS2_PLACEMENT_3D('',#8123,#6604,#6605);
#5663=AXIS2_PLACEMENT_3D('',#8124,#6606,#6607);
#5664=AXIS2_PLACEMENT_3D('',#8126,#6608,#6609);
#5665=AXIS2_PLACEMENT_3D('',#8129,#6611,#6612);
#5666=AXIS2_PLACEMENT_3D('',#8130,#6613,#6614);
#5667=AXIS2_PLACEMENT_3D('',#8139,#6619,#6620);
#5668=AXIS2_PLACEMENT_3D('',#8145,#6624,#6625);
#5669=AXIS2_PLACEMENT_3D('',#8151,#6629,#6630);
#5670=AXIS2_PLACEMENT_3D('',#8154,#6633,#6634);
#5671=AXIS2_PLACEMENT_3D('',#8155,#6635,#6636);
#6415=DIRECTION('axis',(0.,0.,1.));
#6416=DIRECTION('refdir',(1.,0.,0.));
#6417=DIRECTION('center_axis',(1.,0.,0.));
#6418=DIRECTION('ref_axis',(0.,0.,-1.));
#6419=DIRECTION('center_axis',(1.,0.,0.));
#6420=DIRECTION('ref_axis',(0.,0.,-1.));
#6421=DIRECTION('',(1.,0.,0.));
#6422=DIRECTION('center_axis',(-1.,0.,0.));
#6423=DIRECTION('ref_axis',(0.,0.,-1.));
#6424=DIRECTION('center_axis',(1.,0.,0.));
#6425=DIRECTION('ref_axis',(0.,0.,-1.));
#6426=DIRECTION('center_axis',(1.,0.,0.));
#6427=DIRECTION('ref_axis',(0.,0.,-1.));
#6428=DIRECTION('',(1.,0.,0.));
#6429=DIRECTION('center_axis',(-1.,0.,0.));
#6430=DIRECTION('ref_axis',(0.,0.,-1.));
#6431=DIRECTION('center_axis',(1.,0.,0.));
#6432=DIRECTION('ref_axis',(0.,0.,-1.));
#6433=DIRECTION('center_axis',(1.,0.,0.));
#6434=DIRECTION('ref_axis',(0.,0.,-1.));
#6435=DIRECTION('',(1.,0.,0.));
#6436=DIRECTION('center_axis',(-1.,0.,0.));
#6437=DIRECTION('ref_axis',(0.,0.,-1.));
#6438=DIRECTION('center_axis',(1.,0.,0.));
#6439=DIRECTION('ref_axis',(0.,0.,-1.));
#6440=DIRECTION('center_axis',(1.,0.,0.));
#6441=DIRECTION('ref_axis',(0.,0.,-1.));
#6442=DIRECTION('',(1.,0.,0.));
#6443=DIRECTION('center_axis',(-1.,0.,0.));
#6444=DIRECTION('ref_axis',(0.,0.,-1.));
#6445=DIRECTION('center_axis',(1.,0.,0.));
#6446=DIRECTION('ref_axis',(0.,0.,-1.));
#6447=DIRECTION('center_axis',(1.,0.,0.));
#6448=DIRECTION('ref_axis',(0.,0.,-1.));
#6449=DIRECTION('',(1.,0.,0.));
#6450=DIRECTION('center_axis',(-1.,0.,0.));
#6451=DIRECTION('ref_axis',(0.,0.,-1.));
#6452=DIRECTION('center_axis',(1.,0.,0.));
#6453=DIRECTION('ref_axis',(0.,0.,-1.));
#6454=DIRECTION('center_axis',(1.,0.,0.));
#6455=DIRECTION('ref_axis',(0.,0.,-1.));
#6456=DIRECTION('',(1.,0.,0.));
#6457=DIRECTION('center_axis',(-1.,0.,0.));
#6458=DIRECTION('ref_axis',(0.,0.,-1.));
#6459=DIRECTION('center_axis',(1.,0.,0.));
#6460=DIRECTION('ref_axis',(0.,0.,-1.));
#6461=DIRECTION('center_axis',(1.,0.,0.));
#6462=DIRECTION('ref_axis',(0.,0.,-1.));
#6463=DIRECTION('',(1.,0.,0.));
#6464=DIRECTION('center_axis',(-1.,0.,0.));
#6465=DIRECTION('ref_axis',(0.,0.,-1.));
#6466=DIRECTION('center_axis',(1.,0.,0.));
#6467=DIRECTION('ref_axis',(0.,0.,-1.));
#6468=DIRECTION('center_axis',(1.,0.,0.));
#6469=DIRECTION('ref_axis',(0.,0.,-1.));
#6470=DIRECTION('',(1.,0.,0.));
#6471=DIRECTION('center_axis',(-1.,0.,0.));
#6472=DIRECTION('ref_axis',(0.,0.,-1.));
#6473=DIRECTION('center_axis',(1.,0.,0.));
#6474=DIRECTION('ref_axis',(0.,0.,-1.));
#6475=DIRECTION('center_axis',(1.,0.,0.));
#6476=DIRECTION('ref_axis',(0.,0.,-1.));
#6477=DIRECTION('',(1.,0.,0.));
#6478=DIRECTION('center_axis',(-1.,0.,0.));
#6479=DIRECTION('ref_axis',(0.,0.,-1.));
#6480=DIRECTION('center_axis',(1.,0.,0.));
#6481=DIRECTION('ref_axis',(0.,0.,-1.));
#6482=DIRECTION('center_axis',(1.,0.,0.));
#6483=DIRECTION('ref_axis',(0.,0.,-1.));
#6484=DIRECTION('',(1.,0.,0.));
#6485=DIRECTION('center_axis',(-1.,0.,0.));
#6486=DIRECTION('ref_axis',(0.,0.,-1.));
#6487=DIRECTION('center_axis',(1.,0.,0.));
#6488=DIRECTION('ref_axis',(0.,0.,-1.));
#6489=DIRECTION('center_axis',(1.,0.,0.));
#6490=DIRECTION('ref_axis',(0.,0.,-1.));
#6491=DIRECTION('',(1.,0.,0.));
#6492=DIRECTION('center_axis',(-1.,0.,0.));
#6493=DIRECTION('ref_axis',(0.,0.,-1.));
#6494=DIRECTION('center_axis',(1.,0.,0.));
#6495=DIRECTION('ref_axis',(0.,0.,-1.));
#6496=DIRECTION('center_axis',(1.,0.,0.));
#6497=DIRECTION('ref_axis',(0.,0.,-1.));
#6498=DIRECTION('',(1.,0.,0.));
#6499=DIRECTION('center_axis',(-1.,0.,0.));
#6500=DIRECTION('ref_axis',(0.,0.,-1.));
#6501=DIRECTION('center_axis',(1.,0.,0.));
#6502=DIRECTION('ref_axis',(0.,0.,-1.));
#6503=DIRECTION('center_axis',(1.,0.,0.));
#6504=DIRECTION('ref_axis',(0.,0.,-1.));
#6505=DIRECTION('',(1.,0.,0.));
#6506=DIRECTION('center_axis',(-1.,0.,0.));
#6507=DIRECTION('ref_axis',(0.,0.,-1.));
#6508=DIRECTION('center_axis',(1.,0.,0.));
#6509=DIRECTION('ref_axis',(0.,0.,-1.));
#6510=DIRECTION('center_axis',(1.,0.,0.));
#6511=DIRECTION('ref_axis',(0.,0.,-1.));
#6512=DIRECTION('',(1.,0.,0.));
#6513=DIRECTION('center_axis',(-1.,0.,0.));
#6514=DIRECTION('ref_axis',(0.,0.,-1.));
#6515=DIRECTION('center_axis',(1.,0.,0.));
#6516=DIRECTION('ref_axis',(0.,0.,-1.));
#6517=DIRECTION('center_axis',(1.,0.,0.));
#6518=DIRECTION('ref_axis',(0.,0.,-1.));
#6519=DIRECTION('',(1.,0.,0.));
#6520=DIRECTION('center_axis',(-1.,0.,0.));
#6521=DIRECTION('ref_axis',(0.,0.,-1.));
#6522=DIRECTION('center_axis',(1.,0.,0.));
#6523=DIRECTION('ref_axis',(0.,0.,-1.));
#6524=DIRECTION('center_axis',(1.,0.,0.));
#6525=DIRECTION('ref_axis',(0.,0.,-1.));
#6526=DIRECTION('',(1.,0.,0.));
#6527=DIRECTION('center_axis',(-1.,0.,0.));
#6528=DIRECTION('ref_axis',(0.,0.,-1.));
#6529=DIRECTION('center_axis',(1.,0.,0.));
#6530=DIRECTION('ref_axis',(0.,0.,-1.));
#6531=DIRECTION('center_axis',(1.,0.,0.));
#6532=DIRECTION('ref_axis',(0.,0.,-1.));
#6533=DIRECTION('',(1.,0.,0.));
#6534=DIRECTION('center_axis',(-1.,0.,0.));
#6535=DIRECTION('ref_axis',(0.,0.,-1.));
#6536=DIRECTION('center_axis',(1.,0.,0.));
#6537=DIRECTION('ref_axis',(0.,0.,-1.));
#6538=DIRECTION('center_axis',(1.,0.,0.));
#6539=DIRECTION('ref_axis',(0.,0.,-1.));
#6540=DIRECTION('',(1.,0.,0.));
#6541=DIRECTION('center_axis',(-1.,0.,0.));
#6542=DIRECTION('ref_axis',(0.,0.,-1.));
#6543=DIRECTION('center_axis',(1.,0.,0.));
#6544=DIRECTION('ref_axis',(0.,0.,-1.));
#6545=DIRECTION('center_axis',(1.,0.,0.));
#6546=DIRECTION('ref_axis',(0.,0.,-1.));
#6547=DIRECTION('',(1.,0.,0.));
#6548=DIRECTION('center_axis',(-1.,0.,0.));
#6549=DIRECTION('ref_axis',(0.,0.,-1.));
#6550=DIRECTION('center_axis',(1.,0.,0.));
#6551=DIRECTION('ref_axis',(0.,0.,-1.));
#6552=DIRECTION('center_axis',(1.,0.,0.));
#6553=DIRECTION('ref_axis',(0.,0.,-1.));
#6554=DIRECTION('',(1.,0.,0.));
#6555=DIRECTION('center_axis',(-1.,0.,0.));
#6556=DIRECTION('ref_axis',(0.,0.,-1.));
#6557=DIRECTION('center_axis',(1.,0.,0.));
#6558=DIRECTION('ref_axis',(0.,0.,-1.));
#6559=DIRECTION('center_axis',(1.,0.,0.));
#6560=DIRECTION('ref_axis',(0.,0.,-1.));
#6561=DIRECTION('',(1.,0.,0.));
#6562=DIRECTION('center_axis',(-1.,0.,0.));
#6563=DIRECTION('ref_axis',(0.,0.,-1.));
#6564=DIRECTION('center_axis',(1.,0.,0.));
#6565=DIRECTION('ref_axis',(0.,0.,-1.));
#6566=DIRECTION('center_axis',(1.,0.,0.));
#6567=DIRECTION('ref_axis',(0.,0.,-1.));
#6568=DIRECTION('',(1.,0.,0.));
#6569=DIRECTION('center_axis',(-1.,0.,0.));
#6570=DIRECTION('ref_axis',(0.,0.,-1.));
#6571=DIRECTION('center_axis',(1.,0.,0.));
#6572=DIRECTION('ref_axis',(0.,0.,-1.));
#6573=DIRECTION('center_axis',(1.,0.,0.));
#6574=DIRECTION('ref_axis',(0.,0.,-1.));
#6575=DIRECTION('',(1.,0.,0.));
#6576=DIRECTION('center_axis',(-1.,0.,0.));
#6577=DIRECTION('ref_axis',(0.,0.,-1.));
#6578=DIRECTION('center_axis',(1.,0.,0.));
#6579=DIRECTION('ref_axis',(0.,0.,-1.));
#6580=DIRECTION('center_axis',(1.,0.,0.));
#6581=DIRECTION('ref_axis',(0.,0.,-1.));
#6582=DIRECTION('',(1.,0.,0.));
#6583=DIRECTION('center_axis',(-1.,0.,0.));
#6584=DIRECTION('ref_axis',(0.,0.,-1.));
#6585=DIRECTION('center_axis',(1.,0.,0.));
#6586=DIRECTION('ref_axis',(0.,0.,-1.));
#6587=DIRECTION('center_axis',(1.,0.,0.));
#6588=DIRECTION('ref_axis',(0.,0.,-1.));
#6589=DIRECTION('',(1.,0.,0.));
#6590=DIRECTION('center_axis',(-1.,0.,0.));
#6591=DIRECTION('ref_axis',(0.,0.,-1.));
#6592=DIRECTION('center_axis',(1.,0.,0.));
#6593=DIRECTION('ref_axis',(0.,0.,-1.));
#6594=DIRECTION('center_axis',(1.,0.,0.));
#6595=DIRECTION('ref_axis',(0.,0.,-1.));
#6596=DIRECTION('',(1.,0.,0.));
#6597=DIRECTION('center_axis',(-1.,0.,0.));
#6598=DIRECTION('ref_axis',(0.,0.,-1.));
#6599=DIRECTION('center_axis',(1.,0.,0.));
#6600=DIRECTION('ref_axis',(0.,0.,-1.));
#6601=DIRECTION('center_axis',(1.,0.,0.));
#6602=DIRECTION('ref_axis',(0.,0.,-1.));
#6603=DIRECTION('',(1.,0.,0.));
#6604=DIRECTION('center_axis',(-1.,0.,0.));
#6605=DIRECTION('ref_axis',(0.,0.,-1.));
#6606=DIRECTION('center_axis',(1.,0.,0.));
#6607=DIRECTION('ref_axis',(0.,0.,-1.));
#6608=DIRECTION('center_axis',(1.,0.,0.));
#6609=DIRECTION('ref_axis',(0.,0.,-1.));
#6610=DIRECTION('',(1.,0.,0.));
#6611=DIRECTION('center_axis',(-1.,0.,0.));
#6612=DIRECTION('ref_axis',(0.,0.,-1.));
#6613=DIRECTION('center_axis',(0.,1.,0.));
#6614=DIRECTION('ref_axis',(-1.,0.,0.));
#6615=DIRECTION('',(-1.,0.,0.));
#6616=DIRECTION('',(0.,0.,1.));
#6617=DIRECTION('',(-1.,0.,0.));
#6618=DIRECTION('',(0.,0.,1.));
#6619=DIRECTION('center_axis',(1.,0.,0.));
#6620=DIRECTION('ref_axis',(0.,1.,0.));
#6621=DIRECTION('',(0.,1.,0.));
#6622=DIRECTION('',(0.,1.,0.));
#6623=DIRECTION('',(0.,0.,1.));
#6624=DIRECTION('center_axis',(0.,-1.,0.));
#6625=DIRECTION('ref_axis',(1.,0.,0.));
#6626=DIRECTION('',(1.,0.,0.));
#6627=DIRECTION('',(1.,0.,0.));
#6628=DIRECTION('',(0.,0.,1.));
#6629=DIRECTION('center_axis',(-1.,0.,0.));
#6630=DIRECTION('ref_axis',(0.,-1.,0.));
#6631=DIRECTION('',(0.,-1.,0.));
#6632=DIRECTION('',(0.,-1.,0.));
#6633=DIRECTION('center_axis',(0.,0.,1.));
#6634=DIRECTION('ref_axis',(1.,0.,0.));
#6635=DIRECTION('center_axis',(0.,0.,1.));
#6636=DIRECTION('ref_axis',(1.,0.,0.));
#7961=CARTESIAN_POINT('',(0.,0.,0.));
#7962=CARTESIAN_POINT('Origin',(18.7,-2.5,7.));
#7963=CARTESIAN_POINT('',(18.8,-2.5,7.3));
#7964=CARTESIAN_POINT('Origin',(18.8,-2.5,7.));
#7965=CARTESIAN_POINT('',(20.3,-2.5,7.3));
#7966=CARTESIAN_POINT('',(18.7,-2.5,7.3));
#7967=CARTESIAN_POINT('Origin',(20.3,-2.5,7.));
#7968=CARTESIAN_POINT('Origin',(18.7,2.5,7.));
#7969=CARTESIAN_POINT('',(18.8,2.5,7.3));
#7970=CARTESIAN_POINT('Origin',(18.8,2.5,7.));
#7971=CARTESIAN_POINT('',(20.3,2.5,7.3));
#7972=CARTESIAN_POINT('',(18.7,2.5,7.3));
#7973=CARTESIAN_POINT('Origin',(20.3,2.5,7.));
#7974=CARTESIAN_POINT('Origin',(18.7,6.5,-2.));
#7975=CARTESIAN_POINT('',(18.8,6.5,-1.67));
#7976=CARTESIAN_POINT('Origin',(18.8,6.5,-2.));
#7977=CARTESIAN_POINT('',(20.3,6.5,-1.67));
#7978=CARTESIAN_POINT('',(18.7,6.5,-1.67));
#7979=CARTESIAN_POINT('Origin',(20.3,6.5,-2.));
#7980=CARTESIAN_POINT('Origin',(18.7,-6.5,11.));
#7981=CARTESIAN_POINT('',(18.8,-6.5,11.33));
#7982=CARTESIAN_POINT('Origin',(18.8,-6.5,11.));
#7983=CARTESIAN_POINT('',(20.3,-6.5,11.33));
#7984=CARTESIAN_POINT('',(18.7,-6.5,11.33));
#7985=CARTESIAN_POINT('Origin',(20.3,-6.5,11.));
#7986=CARTESIAN_POINT('Origin',(18.7,-6.5,-2.));
#7987=CARTESIAN_POINT('',(18.8,-6.5,-1.67));
#7988=CARTESIAN_POINT('Origin',(18.8,-6.5,-2.));
#7989=CARTESIAN_POINT('',(20.3,-6.5,-1.67));
#7990=CARTESIAN_POINT('',(18.7,-6.5,-1.67));
#7991=CARTESIAN_POINT('Origin',(20.3,-6.5,-2.));
#7992=CARTESIAN_POINT('Origin',(18.7,6.5,11.));
#7993=CARTESIAN_POINT('',(18.8,6.5,11.33));
#7994=CARTESIAN_POINT('Origin',(18.8,6.5,11.));
#7995=CARTESIAN_POINT('',(20.3,6.5,11.33));
#7996=CARTESIAN_POINT('',(18.7,6.5,11.33));
#7997=CARTESIAN_POINT('Origin',(20.3,6.5,11.));
#7998=CARTESIAN_POINT('Origin',(18.7,0.,-0.8));
#7999=CARTESIAN_POINT('',(18.8,-4.04133443718626E-17,-0.47));
#8000=CARTESIAN_POINT('Origin',(18.8,0.,-0.8));
#8001=CARTESIAN_POINT('',(20.3,4.04133443718626E-17,-0.47));
#8002=CARTESIAN_POINT('',(18.7,-4.04133443718626E-17,-0.47));
#8003=CARTESIAN_POINT('Origin',(20.3,0.,-0.8));
#8004=CARTESIAN_POINT('Origin',(18.7,0.,4.));
#8005=CARTESIAN_POINT('',(18.8,-4.04133443718627E-17,4.33));
#8006=CARTESIAN_POINT('Origin',(18.8,0.,4.));
#8007=CARTESIAN_POINT('',(20.3,4.04133443718627E-17,4.33));
#8008=CARTESIAN_POINT('',(18.7,-4.04133443718627E-17,4.33));
#8009=CARTESIAN_POINT('Origin',(20.3,0.,4.));
#8010=CARTESIAN_POINT('Origin',(18.7,5.,7.));
#8011=CARTESIAN_POINT('',(18.8,5.,7.34));
#8012=CARTESIAN_POINT('Origin',(18.8,5.,7.));
#8013=CARTESIAN_POINT('',(20.3,5.,7.34));
#8014=CARTESIAN_POINT('',(18.7,5.,7.34));
#8015=CARTESIAN_POINT('Origin',(20.3,5.,7.));
#8016=CARTESIAN_POINT('Origin',(18.7,5.,2.));
#8017=CARTESIAN_POINT('',(18.8,5.,2.34));
#8018=CARTESIAN_POINT('Origin',(18.8,5.,2.));
#8019=CARTESIAN_POINT('',(20.3,5.,2.34));
#8020=CARTESIAN_POINT('',(18.7,5.,2.34));
#8021=CARTESIAN_POINT('Origin',(20.3,5.,2.));
#8022=CARTESIAN_POINT('Origin',(18.7,2.5,9.5));
#8023=CARTESIAN_POINT('',(18.8,2.5,9.84));
#8024=CARTESIAN_POINT('Origin',(18.8,2.5,9.5));
#8025=CARTESIAN_POINT('',(20.3,2.5,9.84));
#8026=CARTESIAN_POINT('',(18.7,2.5,9.84));
#8027=CARTESIAN_POINT('Origin',(20.3,2.5,9.5));
#8028=CARTESIAN_POINT('Origin',(18.7,2.5,2.));
#8029=CARTESIAN_POINT('',(18.8,2.5,2.34));
#8030=CARTESIAN_POINT('Origin',(18.8,2.5,2.));
#8031=CARTESIAN_POINT('',(20.3,2.5,2.34));
#8032=CARTESIAN_POINT('',(18.7,2.5,2.34));
#8033=CARTESIAN_POINT('Origin',(20.3,2.5,2.));
#8034=CARTESIAN_POINT('Origin',(18.7,0.,9.5));
#8035=CARTESIAN_POINT('',(18.8,-4.163799117101E-17,9.84));
#8036=CARTESIAN_POINT('Origin',(18.8,0.,9.5));
#8037=CARTESIAN_POINT('',(20.3,4.163799117101E-17,9.84));
#8038=CARTESIAN_POINT('',(18.7,-4.163799117101E-17,9.84));
#8039=CARTESIAN_POINT('Origin',(20.3,0.,9.5));
#8040=CARTESIAN_POINT('Origin',(18.7,0.,7.));
#8041=CARTESIAN_POINT('',(18.8,-4.163799117101E-17,7.34));
#8042=CARTESIAN_POINT('Origin',(18.8,0.,7.));
#8043=CARTESIAN_POINT('',(20.3,4.163799117101E-17,7.34));
#8044=CARTESIAN_POINT('',(18.7,-4.163799117101E-17,7.34));
#8045=CARTESIAN_POINT('Origin',(20.3,0.,7.));
#8046=CARTESIAN_POINT('Origin',(18.7,-2.5,4.5));
#8047=CARTESIAN_POINT('',(18.8,-2.5,4.84));
#8048=CARTESIAN_POINT('Origin',(18.8,-2.5,4.5));
#8049=CARTESIAN_POINT('',(20.3,-2.5,4.84));
#8050=CARTESIAN_POINT('',(18.7,-2.5,4.84));
#8051=CARTESIAN_POINT('Origin',(20.3,-2.5,4.5));
#8052=CARTESIAN_POINT('Origin',(18.7,-2.5,-0.5));
#8053=CARTESIAN_POINT('',(18.8,-2.5,-0.16));
#8054=CARTESIAN_POINT('Origin',(18.8,-2.5,-0.5));
#8055=CARTESIAN_POINT('',(20.3,-2.5,-0.16));
#8056=CARTESIAN_POINT('',(18.7,-2.5,-0.16));
#8057=CARTESIAN_POINT('Origin',(20.3,-2.5,-0.5));
#8058=CARTESIAN_POINT('Origin',(18.7,-5.,7.));
#8059=CARTESIAN_POINT('',(18.8,-5.,7.34));
#8060=CARTESIAN_POINT('Origin',(18.8,-5.,7.));
#8061=CARTESIAN_POINT('',(20.3,-5.,7.34));
#8062=CARTESIAN_POINT('',(18.7,-5.,7.34));
#8063=CARTESIAN_POINT('Origin',(20.3,-5.,7.));
#8064=CARTESIAN_POINT('Origin',(18.7,-5.,2.));
#8065=CARTESIAN_POINT('',(18.8,-5.,2.34));
#8066=CARTESIAN_POINT('Origin',(18.8,-5.,2.));
#8067=CARTESIAN_POINT('',(20.3,-5.,2.34));
#8068=CARTESIAN_POINT('',(18.7,-5.,2.34));
#8069=CARTESIAN_POINT('Origin',(20.3,-5.,2.));
#8070=CARTESIAN_POINT('Origin',(18.7,-5.,4.5));
#8071=CARTESIAN_POINT('',(18.8,-5.,4.84));
#8072=CARTESIAN_POINT('Origin',(18.8,-5.,4.5));
#8073=CARTESIAN_POINT('',(20.3,-5.,4.84));
#8074=CARTESIAN_POINT('',(18.7,-5.,4.84));
#8075=CARTESIAN_POINT('Origin',(20.3,-5.,4.5));
#8076=CARTESIAN_POINT('Origin',(18.7,-5.,9.5));
#8077=CARTESIAN_POINT('',(18.8,-5.,9.84));
#8078=CARTESIAN_POINT('Origin',(18.8,-5.,9.5));
#8079=CARTESIAN_POINT('',(20.3,-5.,9.84));
#8080=CARTESIAN_POINT('',(18.7,-5.,9.84));
#8081=CARTESIAN_POINT('Origin',(20.3,-5.,9.5));
#8082=CARTESIAN_POINT('Origin',(18.7,-2.5,2.));
#8083=CARTESIAN_POINT('',(18.8,-2.5,2.34));
#8084=CARTESIAN_POINT('Origin',(18.8,-2.5,2.));
#8085=CARTESIAN_POINT('',(20.3,-2.5,2.34));
#8086=CARTESIAN_POINT('',(18.7,-2.5,2.34));
#8087=CARTESIAN_POINT('Origin',(20.3,-2.5,2.));
#8088=CARTESIAN_POINT('Origin',(18.7,-2.5,9.5));
#8089=CARTESIAN_POINT('',(18.8,-2.5,9.84));
#8090=CARTESIAN_POINT('Origin',(18.8,-2.5,9.5));
#8091=CARTESIAN_POINT('',(20.3,-2.5,9.84));
#8092=CARTESIAN_POINT('',(18.7,-2.5,9.84));
#8093=CARTESIAN_POINT('Origin',(20.3,-2.5,9.5));
#8094=CARTESIAN_POINT('Origin',(18.7,-5.,-0.5));
#8095=CARTESIAN_POINT('',(18.8,-5.,-0.16));
#8096=CARTESIAN_POINT('Origin',(18.8,-5.,-0.5));
#8097=CARTESIAN_POINT('',(20.3,-5.,-0.16));
#8098=CARTESIAN_POINT('',(18.7,-5.,-0.16));
#8099=CARTESIAN_POINT('Origin',(20.3,-5.,-0.5));
#8100=CARTESIAN_POINT('Origin',(18.7,2.5,-0.5));
#8101=CARTESIAN_POINT('',(18.8,2.5,-0.16));
#8102=CARTESIAN_POINT('Origin',(18.8,2.5,-0.5));
#8103=CARTESIAN_POINT('',(20.3,2.5,-0.16));
#8104=CARTESIAN_POINT('',(18.7,2.5,-0.16));
#8105=CARTESIAN_POINT('Origin',(20.3,2.5,-0.5));
#8106=CARTESIAN_POINT('Origin',(18.7,2.5,4.5));
#8107=CARTESIAN_POINT('',(18.8,2.5,4.84));
#8108=CARTESIAN_POINT('Origin',(18.8,2.5,4.5));
#8109=CARTESIAN_POINT('',(20.3,2.5,4.84));
#8110=CARTESIAN_POINT('',(18.7,2.5,4.84));
#8111=CARTESIAN_POINT('Origin',(20.3,2.5,4.5));
#8112=CARTESIAN_POINT('Origin',(18.7,5.,-0.5));
#8113=CARTESIAN_POINT('',(18.8,5.,-0.16));
#8114=CARTESIAN_POINT('Origin',(18.8,5.,-0.5));
#8115=CARTESIAN_POINT('',(20.3,5.,-0.16));
#8116=CARTESIAN_POINT('',(18.7,5.,-0.16));
#8117=CARTESIAN_POINT('Origin',(20.3,5.,-0.5));
#8118=CARTESIAN_POINT('Origin',(18.7,5.,4.5));
#8119=CARTESIAN_POINT('',(18.8,5.,4.84));
#8120=CARTESIAN_POINT('Origin',(18.8,5.,4.5));
#8121=CARTESIAN_POINT('',(20.3,5.,4.84));
#8122=CARTESIAN_POINT('',(18.7,5.,4.84));
#8123=CARTESIAN_POINT('Origin',(20.3,5.,4.5));
#8124=CARTESIAN_POINT('Origin',(18.7,5.,9.5));
#8125=CARTESIAN_POINT('',(18.8,5.,9.84));
#8126=CARTESIAN_POINT('Origin',(18.8,5.,9.5));
#8127=CARTESIAN_POINT('',(20.3,5.,9.84));
#8128=CARTESIAN_POINT('',(18.7,5.,9.84));
#8129=CARTESIAN_POINT('Origin',(20.3,5.,9.5));
#8130=CARTESIAN_POINT('Origin',(20.3,7.5,-3.));
#8131=CARTESIAN_POINT('',(20.3,7.5,-3.));
#8132=CARTESIAN_POINT('',(18.8,7.5,-3.));
#8133=CARTESIAN_POINT('',(20.3,7.5,-3.));
#8134=CARTESIAN_POINT('',(18.8,7.5,12.));
#8135=CARTESIAN_POINT('',(18.8,7.5,-3.));
#8136=CARTESIAN_POINT('',(20.3,7.5,12.));
#8137=CARTESIAN_POINT('',(20.3,7.5,12.));
#8138=CARTESIAN_POINT('',(20.3,7.5,-3.));
#8139=CARTESIAN_POINT('Origin',(20.3,-7.5,-3.));
#8140=CARTESIAN_POINT('',(20.3,-7.5,-3.));
#8141=CARTESIAN_POINT('',(20.3,-7.5,-3.));
#8142=CARTESIAN_POINT('',(20.3,-7.5,12.));
#8143=CARTESIAN_POINT('',(20.3,-7.5,12.));
#8144=CARTESIAN_POINT('',(20.3,-7.5,-3.));
#8145=CARTESIAN_POINT('Origin',(18.8,-7.5,-3.));
#8146=CARTESIAN_POINT('',(18.8,-7.5,-3.));
#8147=CARTESIAN_POINT('',(18.8,-7.5,-3.));
#8148=CARTESIAN_POINT('',(18.8,-7.5,12.));
#8149=CARTESIAN_POINT('',(18.8,-7.5,12.));
#8150=CARTESIAN_POINT('',(18.8,-7.5,-3.));
#8151=CARTESIAN_POINT('Origin',(18.8,7.5,-3.));
#8152=CARTESIAN_POINT('',(18.8,7.5,-3.));
#8153=CARTESIAN_POINT('',(18.8,7.5,12.));
#8154=CARTESIAN_POINT('Origin',(19.55,0.,12.));
#8155=CARTESIAN_POINT('Origin',(19.55,0.,-3.));
#9232=UNCERTAINTY_MEASURE_WITH_UNIT(LENGTH_MEASURE(0.001),#9286,
'DISTANCE_ACCURACY_VALUE',
'Maximum model space distance between geometric entities at asserted c
onnectivities');
#9255=UNCERTAINTY_MEASURE_WITH_UNIT(LENGTH_MEASURE(0.001),#9286,
'DISTANCE_ACCURACY_VALUE',
'Maximum model space distance between geometric entities at asserted c
onnectivities');
#9262=(
GEOMETRIC_REPRESENTATION_CONTEXT(3)
GLOBAL_UNCERTAINTY_ASSIGNED_CONTEXT((#9232))
GLOBAL_UNIT_ASSIGNED_CONTEXT((#9286,#9288,#9289))
REPRESENTATION_CONTEXT('','3D')
);
#9285=(
GEOMETRIC_REPRESENTATION_CONTEXT(3)
GLOBAL_UNCERTAINTY_ASSIGNED_CONTEXT((#9255))
GLOBAL_UNIT_ASSIGNED_CONTEXT((#9286,#9288,#9289))
REPRESENTATION_CONTEXT('','3D')
);
#9286=(
LENGTH_UNIT()
NAMED_UNIT(*)
SI_UNIT(.CENTI.,.METRE.)
);
#9288=(
NAMED_UNIT(*)
PLANE_ANGLE_UNIT()
SI_UNIT($,.RADIAN.)
);
#9289=(
NAMED_UNIT(*)
SI_UNIT($,.STERADIAN.)
SOLID_ANGLE_UNIT()
);
#9296=SHAPE_DEFINITION_REPRESENTATION(#9325,#9400);
#9325=PRODUCT_DEFINITION_SHAPE('',$,#9430);
#9400=SHAPE_REPRESENTATION('',(#5581),#9262);
#9423=PRODUCT_DEFINITION_CONTEXT('part definition',#9512,'design');
#9430=PRODUCT_DEFINITION('Located grid plate','Located grid plate',#9459,
#9423);
#9459=PRODUCT_DEFINITION_FORMATION('',$,#9520);
#9512=APPLICATION_CONTEXT(
'Core Data for Automotive Mechanical Design Process');
#9513=PRODUCT_CONTEXT('part definition',#9512,'mechanical');
#9520=PRODUCT('Located grid plate','Located grid plate',
'Located grid plate',(#9513));
#9592=COLOUR_RGB('Light Blue',0.38,0.62,0.78);
#9593=FILL_AREA_STYLE_COLOUR('',#9592);
#9594=FILL_AREA_STYLE('',(#9593));
#9595=SURFACE_STYLE_FILL_AREA(#9594);
#9596=SURFACE_SIDE_STYLE('',(#9595));
#9597=SURFACE_STYLE_USAGE(.BOTH.,#9596);
#9598=PRESENTATION_STYLE_ASSIGNMENT((#9597));
ENDSEC;
END-ISO-10303-21;
